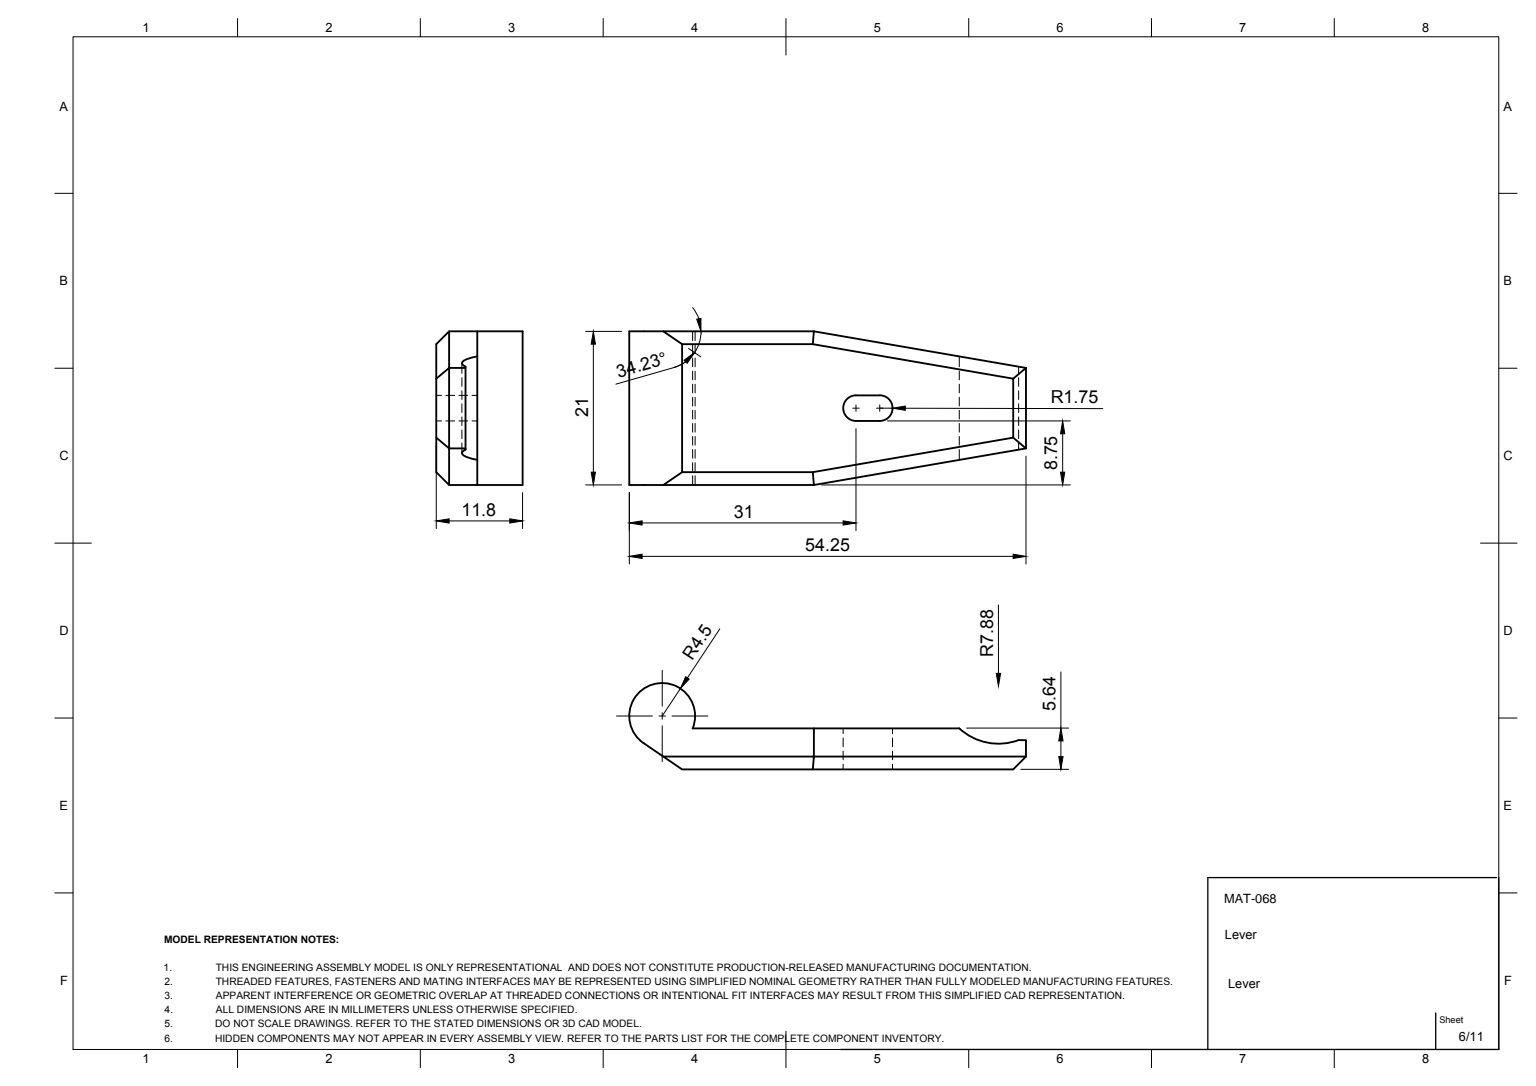
ISO-10303-21;
HEADER;
/* Generated by software containing ST-Developer
 * from STEP Tools, Inc. (www.steptools.com) 
 */

FILE_DESCRIPTION(
/* description */ ('CAx-IF Rec.Pracs.---Representation and Presentation of Product Manufa
cturing Information (PMI)---4.0---2014-10-13'),
/* implementation_level */ '2;1');

FILE_NAME(
/* name */ 'Lever.step',
/* time_stamp */ '2026-10-24T16:53:48-07:00',
/* author */ (''),
/* organization */ (''),
/* preprocessor_version */ 'ST-DEVELOPER v20.2',
/* originating_system */ 'Autodesk Translation Framework v15.17.0.0',
/* authorisation */ '');

FILE_SCHEMA (('AP242_MANAGED_MODEL_BASED_3D_ENGINEERING_MIM_LF { 1 0 10303 442 2 1 4 }'));
ENDSEC;

DATA;
#10=MECHANICAL_DESIGN_GEOMETRIC_PRESENTATION_REPRESENTATION('',(#3493),#107910);
#884=ELLIPSE('',#45698,0.00800033336362062,0.00788400944250588);
#885=ELLIPSE('',#45699,0.00800033336362222,0.0078840094425091);
#3473=SHAPE_REPRESENTATION_RELATIONSHIP('SRR','None',#107951,#3483);
#3483=ADVANCED_BREP_SHAPE_REPRESENTATION('',(#3503),#107904);
#3493=STYLED_ITEM('',(#108006),#3503);
#3503=MANIFOLD_SOLID_BREP('Body1',#45541);
#3511=FACE_BOUND('',#6702,.T.);
#3512=FACE_BOUND('',#6707,.T.);
#3550=PLANE('',#45695);
#3551=PLANE('',#45700);
#3552=PLANE('',#45701);
#3553=PLANE('',#45702);
#3554=PLANE('',#45704);
#3555=PLANE('',#45705);
#3556=PLANE('',#45706);
#3557=PLANE('',#45707);
#3558=PLANE('',#45708);
#3559=PLANE('',#45710);
#3560=PLANE('',#45711);
#3561=PLANE('',#45712);
#3562=PLANE('',#45713);
#3563=PLANE('',#45714);
#3564=PLANE('',#45715);
#3565=PLANE('',#45716);
#3773=FACE_OUTER_BOUND('',#6699,.T.);
#3774=FACE_OUTER_BOUND('',#6700,.T.);
#3775=FACE_OUTER_BOUND('',#6701,.T.);
#3776=FACE_OUTER_BOUND('',#6703,.T.);
#3777=FACE_OUTER_BOUND('',#6704,.T.);
#3778=FACE_OUTER_BOUND('',#6705,.T.);
#3779=FACE_OUTER_BOUND('',#6706,.T.);
#3780=FACE_OUTER_BOUND('',#6708,.T.);
#3781=FACE_OUTER_BOUND('',#6709,.T.);
#3782=FACE_OUTER_BOUND('',#6710,.T.);
#3783=FACE_OUTER_BOUND('',#6711,.T.);
#3784=FACE_OUTER_BOUND('',#6712,.T.);
#3785=FACE_OUTER_BOUND('',#6713,.T.);
#3786=FACE_OUTER_BOUND('',#6714,.T.);
#3787=FACE_OUTER_BOUND('',#6715,.T.);
#3788=FACE_OUTER_BOUND('',#6716,.T.);
#3789=FACE_OUTER_BOUND('',#6717,.T.);
#3790=FACE_OUTER_BOUND('',#6718,.T.);
#3791=FACE_OUTER_BOUND('',#6719,.T.);
#3792=FACE_OUTER_BOUND('',#6720,.T.);
#6699=EDGE_LOOP('',(#28164,#28165,#28166,#28167));
#6700=EDGE_LOOP('',(#28168,#28169,#28170,#28171));
#6701=EDGE_LOOP('',(#28172,#28173,#28174,#28175,#28176,#28177));
#6702=EDGE_LOOP('',(#28178,#28179,#28180,#28181));
#6703=EDGE_LOOP('',(#28182,#28183,#28184,#28185));
#6704=EDGE_LOOP('',(#28186,#28187,#28188,#28189));
#6705=EDGE_LOOP('',(#28190,#28191,#28192,#28193));
#6706=EDGE_LOOP('',(#28194,#28195,#28196,#28197,#28198,#28199));
#6707=EDGE_LOOP('',(#28200,#28201,#28202,#28203));
#6708=EDGE_LOOP('',(#28204,#28205,#28206,#28207,#28208,#28209));
#6709=EDGE_LOOP('',(#28210,#28211,#28212,#28213,#28214));
#6710=EDGE_LOOP('',(#28215,#28216,#28217,#28218,#28219));
#6711=EDGE_LOOP('',(#28220,#28221,#28222,#28223,#28224,#28225));
#6712=EDGE_LOOP('',(#28226,#28227,#28228,#28229,#28230,#28231));
#6713=EDGE_LOOP('',(#28232,#28233,#28234,#28235));
#6714=EDGE_LOOP('',(#28236,#28237,#28238,#28239));
#6715=EDGE_LOOP('',(#28240,#28241,#28242,#28243));
#6716=EDGE_LOOP('',(#28244,#28245,#28246,#28247));
#6717=EDGE_LOOP('',(#28248,#28249,#28250,#28251));
#6718=EDGE_LOOP('',(#28252,#28253,#28254,#28255));
#6719=EDGE_LOOP('',(#28256,#28257,#28258,#28259));
#6720=EDGE_LOOP('',(#28260,#28261,#28262,#28263));
#9644=LINE('',#63425,#11628);
#9645=LINE('',#63428,#11629);
#9646=LINE('',#63434,#11630);
#9647=LINE('',#63437,#11631);
#9648=LINE('',#63440,#11632);
#9649=LINE('',#63442,#11633);
#9650=LINE('',#63444,#11634);
#9651=LINE('',#63446,#11635);
#9652=LINE('',#63447,#11636);
#9653=LINE('',#63449,#11637);
#9654=LINE('',#63452,#11638);
#9655=LINE('',#63457,#11639);
#9656=LINE('',#63461,#11640);
#9657=LINE('',#63463,#11641);
#9658=LINE('',#63464,#11642);
#9659=LINE('',#63467,#11643);
#9660=LINE('',#63469,#11644);
#9661=LINE('',#63470,#11645);
#9662=LINE('',#63474,#11646);
#9663=LINE('',#63476,#11647);
#9664=LINE('',#63478,#11648);
#9665=LINE('',#63480,#11649);
#9666=LINE('',#63482,#11650);
#9667=LINE('',#63483,#11651);
#9668=LINE('',#63485,#11652);
#9669=LINE('',#63488,#11653);
#9670=LINE('',#63491,#11654);
#9671=LINE('',#63492,#11655);
#9672=LINE('',#63494,#11656);
#9673=LINE('',#63495,#11657);
#9674=LINE('',#63498,#11658);
#9675=LINE('',#63499,#11659);
#9676=LINE('',#63502,#11660);
#9677=LINE('',#63503,#11661);
#9678=LINE('',#63505,#11662);
#9679=LINE('',#63507,#11663);
#9680=LINE('',#63509,#11664);
#9681=LINE('',#63510,#11665);
#9682=LINE('',#63514,#11666);
#9683=LINE('',#63516,#11667);
#9684=LINE('',#63518,#11668);
#9685=LINE('',#63520,#11669);
#11628=VECTOR('',#50447,1.);
#11629=VECTOR('',#50450,1.);
#11630=VECTOR('',#50455,1.);
#11631=VECTOR('',#50458,1.);
#11632=VECTOR('',#50461,1.);
#11633=VECTOR('',#50462,1.);
#11634=VECTOR('',#50463,1.);
#11635=VECTOR('',#50464,1.);
#11636=VECTOR('',#50465,1.);
#11637=VECTOR('',#50466,1.);
#11638=VECTOR('',#50469,1.);
#11639=VECTOR('',#50474,1.);
#11640=VECTOR('',#50479,1.);
#11641=VECTOR('',#50480,1.);
#11642=VECTOR('',#50481,1.);
#11643=VECTOR('',#50484,1.);
#11644=VECTOR('',#50485,1.);
#11645=VECTOR('',#50486,1.);
#11646=VECTOR('',#50489,1.);
#11647=VECTOR('',#50490,1.);
#11648=VECTOR('',#50491,1.);
#11649=VECTOR('',#50492,1.);
#11650=VECTOR('',#50493,1.);
#11651=VECTOR('',#50494,1.);
#11652=VECTOR('',#50495,1.);
#11653=VECTOR('',#50498,1.);
#11654=VECTOR('',#50501,1.);
#11655=VECTOR('',#50502,1.);
#11656=VECTOR('',#50503,1.);
#11657=VECTOR('',#50504,1.);
#11658=VECTOR('',#50507,1.);
#11659=VECTOR('',#50508,1.);
#11660=VECTOR('',#50511,1.);
#11661=VECTOR('',#50512,1.);
#11662=VECTOR('',#50515,1.);
#11663=VECTOR('',#50518,1.);
#11664=VECTOR('',#50521,1.);
#11665=VECTOR('',#50522,1.);
#11666=VECTOR('',#50529,1.);
#11667=VECTOR('',#50532,1.);
#11668=VECTOR('',#50535,1.);
#11669=VECTOR('',#50538,1.);
#13618=CIRCLE('',#45690,0.00175000000001001);
#13619=CIRCLE('',#45691,0.00175000000001001);
#13620=CIRCLE('',#45693,0.00450000000001);
#13621=CIRCLE('',#45694,0.00450000000001);
#13622=CIRCLE('',#45696,0.00175000000001001);
#13623=CIRCLE('',#45703,0.00175000000001001);
#17193=VERTEX_POINT('',#63421);
#17194=VERTEX_POINT('',#63422);
#17195=VERTEX_POINT('',#63424);
#17196=VERTEX_POINT('',#63426);
#17197=VERTEX_POINT('',#63430);
#17198=VERTEX_POINT('',#63431);
#17199=VERTEX_POINT('',#63433);
#17200=VERTEX_POINT('',#63435);
#17201=VERTEX_POINT('',#63439);
#17202=VERTEX_POINT('',#63441);
#17203=VERTEX_POINT('',#63443);
#17204=VERTEX_POINT('',#63445);
#17205=VERTEX_POINT('',#63448);
#17206=VERTEX_POINT('',#63450);
#17207=VERTEX_POINT('',#63454);
#17208=VERTEX_POINT('',#63456);
#17209=VERTEX_POINT('',#63460);
#17210=VERTEX_POINT('',#63462);
#17211=VERTEX_POINT('',#63466);
#17212=VERTEX_POINT('',#63468);
#17213=VERTEX_POINT('',#63472);
#17214=VERTEX_POINT('',#63473);
#17215=VERTEX_POINT('',#63475);
#17216=VERTEX_POINT('',#63477);
#17217=VERTEX_POINT('',#63479);
#17218=VERTEX_POINT('',#63481);
#17219=VERTEX_POINT('',#63484);
#17220=VERTEX_POINT('',#63486);
#17221=VERTEX_POINT('',#63490);
#17222=VERTEX_POINT('',#63493);
#17223=VERTEX_POINT('',#63497);
#17224=VERTEX_POINT('',#63501);
#21224=EDGE_CURVE('',#17193,#17194,#13618,.T.);
#21225=EDGE_CURVE('',#17194,#17195,#9644,.T.);
#21226=EDGE_CURVE('',#17195,#17196,#13619,.T.);
#21227=EDGE_CURVE('',#17193,#17196,#9645,.T.);
#21228=EDGE_CURVE('',#17197,#17198,#13620,.T.);
#21229=EDGE_CURVE('',#17197,#17199,#9646,.T.);
#21230=EDGE_CURVE('',#17199,#17200,#13621,.T.);
#21231=EDGE_CURVE('',#17198,#17200,#9647,.T.);
#21232=EDGE_CURVE('',#17200,#17201,#9648,.T.);
#21233=EDGE_CURVE('',#17202,#17201,#9649,.T.);
#21234=EDGE_CURVE('',#17203,#17202,#9650,.T.);
#21235=EDGE_CURVE('',#17204,#17203,#9651,.T.);
#21236=EDGE_CURVE('',#17198,#17204,#9652,.T.);
#21237=EDGE_CURVE('',#17205,#17193,#9653,.T.);
#21238=EDGE_CURVE('',#17206,#17205,#13622,.T.);
#21239=EDGE_CURVE('',#17194,#17206,#9654,.T.);
#21240=EDGE_CURVE('',#17202,#17207,#884,.T.);
#21241=EDGE_CURVE('',#17208,#17207,#9655,.T.);
#21242=EDGE_CURVE('',#17208,#17203,#885,.T.);
#21243=EDGE_CURVE('',#17207,#17209,#9656,.T.);
#21244=EDGE_CURVE('',#17210,#17209,#9657,.T.);
#21245=EDGE_CURVE('',#17210,#17208,#9658,.T.);
#21246=EDGE_CURVE('',#17209,#17211,#9659,.T.);
#21247=EDGE_CURVE('',#17211,#17212,#9660,.T.);
#21248=EDGE_CURVE('',#17210,#17212,#9661,.T.);
#21249=EDGE_CURVE('',#17213,#17214,#9662,.T.);
#21250=EDGE_CURVE('',#17214,#17215,#9663,.T.);
#21251=EDGE_CURVE('',#17216,#17215,#9664,.T.);
#21252=EDGE_CURVE('',#17216,#17217,#9665,.T.);
#21253=EDGE_CURVE('',#17217,#17218,#9666,.T.);
#21254=EDGE_CURVE('',#17218,#17213,#9667,.T.);
#21255=EDGE_CURVE('',#17219,#17195,#9668,.T.);
#21256=EDGE_CURVE('',#17220,#17219,#13623,.T.);
#21257=EDGE_CURVE('',#17196,#17220,#9669,.T.);
#21258=EDGE_CURVE('',#17215,#17221,#9670,.T.);
#21259=EDGE_CURVE('',#17221,#17199,#9671,.T.);
#21260=EDGE_CURVE('',#17222,#17197,#9672,.T.);
#21261=EDGE_CURVE('',#17222,#17216,#9673,.T.);
#21262=EDGE_CURVE('',#17204,#17223,#9674,.T.);
#21263=EDGE_CURVE('',#17223,#17222,#9675,.T.);
#21264=EDGE_CURVE('',#17221,#17224,#9676,.T.);
#21265=EDGE_CURVE('',#17201,#17224,#9677,.T.);
#21266=EDGE_CURVE('',#17224,#17211,#9678,.T.);
#21267=EDGE_CURVE('',#17212,#17223,#9679,.T.);
#21268=EDGE_CURVE('',#17205,#17220,#9680,.T.);
#21269=EDGE_CURVE('',#17206,#17219,#9681,.T.);
#21270=EDGE_CURVE('',#17217,#17223,#9682,.T.);
#21271=EDGE_CURVE('',#17218,#17212,#9683,.T.);
#21272=EDGE_CURVE('',#17213,#17211,#9684,.T.);
#21273=EDGE_CURVE('',#17214,#17224,#9685,.T.);
#28164=ORIENTED_EDGE('',*,*,#21224,.T.);
#28165=ORIENTED_EDGE('',*,*,#21225,.T.);
#28166=ORIENTED_EDGE('',*,*,#21226,.T.);
#28167=ORIENTED_EDGE('',*,*,#21227,.F.);
#28168=ORIENTED_EDGE('',*,*,#21228,.F.);
#28169=ORIENTED_EDGE('',*,*,#21229,.T.);
#28170=ORIENTED_EDGE('',*,*,#21230,.T.);
#28171=ORIENTED_EDGE('',*,*,#21231,.F.);
#28172=ORIENTED_EDGE('',*,*,#21232,.T.);
#28173=ORIENTED_EDGE('',*,*,#21233,.F.);
#28174=ORIENTED_EDGE('',*,*,#21234,.F.);
#28175=ORIENTED_EDGE('',*,*,#21235,.F.);
#28176=ORIENTED_EDGE('',*,*,#21236,.F.);
#28177=ORIENTED_EDGE('',*,*,#21231,.T.);
#28178=ORIENTED_EDGE('',*,*,#21237,.F.);
#28179=ORIENTED_EDGE('',*,*,#21238,.F.);
#28180=ORIENTED_EDGE('',*,*,#21239,.F.);
#28181=ORIENTED_EDGE('',*,*,#21224,.F.);
#28182=ORIENTED_EDGE('',*,*,#21234,.T.);
#28183=ORIENTED_EDGE('',*,*,#21240,.T.);
#28184=ORIENTED_EDGE('',*,*,#21241,.F.);
#28185=ORIENTED_EDGE('',*,*,#21242,.T.);
#28186=ORIENTED_EDGE('',*,*,#21241,.T.);
#28187=ORIENTED_EDGE('',*,*,#21243,.T.);
#28188=ORIENTED_EDGE('',*,*,#21244,.F.);
#28189=ORIENTED_EDGE('',*,*,#21245,.T.);
#28190=ORIENTED_EDGE('',*,*,#21246,.T.);
#28191=ORIENTED_EDGE('',*,*,#21247,.T.);
#28192=ORIENTED_EDGE('',*,*,#21248,.F.);
#28193=ORIENTED_EDGE('',*,*,#21244,.T.);
#28194=ORIENTED_EDGE('',*,*,#21249,.T.);
#28195=ORIENTED_EDGE('',*,*,#21250,.T.);
#28196=ORIENTED_EDGE('',*,*,#21251,.F.);
#28197=ORIENTED_EDGE('',*,*,#21252,.T.);
#28198=ORIENTED_EDGE('',*,*,#21253,.T.);
#28199=ORIENTED_EDGE('',*,*,#21254,.T.);
#28200=ORIENTED_EDGE('',*,*,#21255,.F.);
#28201=ORIENTED_EDGE('',*,*,#21256,.F.);
#28202=ORIENTED_EDGE('',*,*,#21257,.F.);
#28203=ORIENTED_EDGE('',*,*,#21226,.F.);
#28204=ORIENTED_EDGE('',*,*,#21251,.T.);
#28205=ORIENTED_EDGE('',*,*,#21258,.T.);
#28206=ORIENTED_EDGE('',*,*,#21259,.T.);
#28207=ORIENTED_EDGE('',*,*,#21229,.F.);
#28208=ORIENTED_EDGE('',*,*,#21260,.F.);
#28209=ORIENTED_EDGE('',*,*,#21261,.T.);
#28210=ORIENTED_EDGE('',*,*,#21262,.T.);
#28211=ORIENTED_EDGE('',*,*,#21263,.T.);
#28212=ORIENTED_EDGE('',*,*,#21260,.T.);
#28213=ORIENTED_EDGE('',*,*,#21228,.T.);
#28214=ORIENTED_EDGE('',*,*,#21236,.T.);
#28215=ORIENTED_EDGE('',*,*,#21259,.F.);
#28216=ORIENTED_EDGE('',*,*,#21264,.T.);
#28217=ORIENTED_EDGE('',*,*,#21265,.F.);
#28218=ORIENTED_EDGE('',*,*,#21232,.F.);
#28219=ORIENTED_EDGE('',*,*,#21230,.F.);
#28220=ORIENTED_EDGE('',*,*,#21265,.T.);
#28221=ORIENTED_EDGE('',*,*,#21266,.T.);
#28222=ORIENTED_EDGE('',*,*,#21246,.F.);
#28223=ORIENTED_EDGE('',*,*,#21243,.F.);
#28224=ORIENTED_EDGE('',*,*,#21240,.F.);
#28225=ORIENTED_EDGE('',*,*,#21233,.T.);
#28226=ORIENTED_EDGE('',*,*,#21248,.T.);
#28227=ORIENTED_EDGE('',*,*,#21267,.T.);
#28228=ORIENTED_EDGE('',*,*,#21262,.F.);
#28229=ORIENTED_EDGE('',*,*,#21235,.T.);
#28230=ORIENTED_EDGE('',*,*,#21242,.F.);
#28231=ORIENTED_EDGE('',*,*,#21245,.F.);
#28232=ORIENTED_EDGE('',*,*,#21238,.T.);
#28233=ORIENTED_EDGE('',*,*,#21268,.T.);
#28234=ORIENTED_EDGE('',*,*,#21256,.T.);
#28235=ORIENTED_EDGE('',*,*,#21269,.F.);
#28236=ORIENTED_EDGE('',*,*,#21237,.T.);
#28237=ORIENTED_EDGE('',*,*,#21227,.T.);
#28238=ORIENTED_EDGE('',*,*,#21257,.T.);
#28239=ORIENTED_EDGE('',*,*,#21268,.F.);
#28240=ORIENTED_EDGE('',*,*,#21239,.T.);
#28241=ORIENTED_EDGE('',*,*,#21269,.T.);
#28242=ORIENTED_EDGE('',*,*,#21255,.T.);
#28243=ORIENTED_EDGE('',*,*,#21225,.F.);
#28244=ORIENTED_EDGE('',*,*,#21261,.F.);
#28245=ORIENTED_EDGE('',*,*,#21263,.F.);
#28246=ORIENTED_EDGE('',*,*,#21270,.F.);
#28247=ORIENTED_EDGE('',*,*,#21252,.F.);
#28248=ORIENTED_EDGE('',*,*,#21270,.T.);
#28249=ORIENTED_EDGE('',*,*,#21267,.F.);
#28250=ORIENTED_EDGE('',*,*,#21271,.F.);
#28251=ORIENTED_EDGE('',*,*,#21253,.F.);
#28252=ORIENTED_EDGE('',*,*,#21271,.T.);
#28253=ORIENTED_EDGE('',*,*,#21247,.F.);
#28254=ORIENTED_EDGE('',*,*,#21272,.F.);
#28255=ORIENTED_EDGE('',*,*,#21254,.F.);
#28256=ORIENTED_EDGE('',*,*,#21272,.T.);
#28257=ORIENTED_EDGE('',*,*,#21266,.F.);
#28258=ORIENTED_EDGE('',*,*,#21273,.F.);
#28259=ORIENTED_EDGE('',*,*,#21249,.F.);
#28260=ORIENTED_EDGE('',*,*,#21273,.T.);
#28261=ORIENTED_EDGE('',*,*,#21264,.F.);
#28262=ORIENTED_EDGE('',*,*,#21258,.F.);
#28263=ORIENTED_EDGE('',*,*,#21250,.F.);
#41965=CYLINDRICAL_SURFACE('',#45689,0.00175);
#41966=CYLINDRICAL_SURFACE('',#45692,0.0045);
#41967=CYLINDRICAL_SURFACE('',#45697,0.00788400944250797);
#41968=CYLINDRICAL_SURFACE('',#45709,0.00175);
#42628=ADVANCED_FACE('',(#3773),#41965,.F.);
#42629=ADVANCED_FACE('',(#3774),#41966,.T.);
#42630=ADVANCED_FACE('',(#3775,#3511),#3550,.F.);
#42631=ADVANCED_FACE('',(#3776),#41967,.F.);
#42632=ADVANCED_FACE('',(#3777),#3551,.F.);
#42633=ADVANCED_FACE('',(#3778),#3552,.F.);
#42634=ADVANCED_FACE('',(#3779,#3512),#3553,.F.);
#42635=ADVANCED_FACE('',(#3780),#3554,.F.);
#42636=ADVANCED_FACE('',(#3781),#3555,.T.);
#42637=ADVANCED_FACE('',(#3782),#3556,.T.);
#42638=ADVANCED_FACE('',(#3783),#3557,.F.);
#42639=ADVANCED_FACE('',(#3784),#3558,.F.);
#42640=ADVANCED_FACE('',(#3785),#41968,.F.);
#42641=ADVANCED_FACE('',(#3786),#3559,.F.);
#42642=ADVANCED_FACE('',(#3787),#3560,.F.);
#42643=ADVANCED_FACE('',(#3788),#3561,.T.);
#42644=ADVANCED_FACE('',(#3789),#3562,.F.);
#42645=ADVANCED_FACE('',(#3790),#3563,.F.);
#42646=ADVANCED_FACE('',(#3791),#3564,.F.);
#42647=ADVANCED_FACE('',(#3792),#3565,.T.);
#45541=CLOSED_SHELL('',(#42628,#42629,#42630,#42631,#42632,#42633,#42634,
#42635,#42636,#42637,#42638,#42639,#42640,#42641,#42642,#42643,#42644,#42645,
#42646,#42647));
#45688=AXIS2_PLACEMENT_3D('',#63419,#50441,#50442);
#45689=AXIS2_PLACEMENT_3D('',#63420,#50443,#50444);
#45690=AXIS2_PLACEMENT_3D('',#63423,#50445,#50446);
#45691=AXIS2_PLACEMENT_3D('',#63427,#50448,#50449);
#45692=AXIS2_PLACEMENT_3D('',#63429,#50451,#50452);
#45693=AXIS2_PLACEMENT_3D('',#63432,#50453,#50454);
#45694=AXIS2_PLACEMENT_3D('',#63436,#50456,#50457);
#45695=AXIS2_PLACEMENT_3D('',#63438,#50459,#50460);
#45696=AXIS2_PLACEMENT_3D('',#63451,#50467,#50468);
#45697=AXIS2_PLACEMENT_3D('',#63453,#50470,#50471);
#45698=AXIS2_PLACEMENT_3D('',#63455,#50472,#50473);
#45699=AXIS2_PLACEMENT_3D('',#63458,#50475,#50476);
#45700=AXIS2_PLACEMENT_3D('',#63459,#50477,#50478);
#45701=AXIS2_PLACEMENT_3D('',#63465,#50482,#50483);
#45702=AXIS2_PLACEMENT_3D('',#63471,#50487,#50488);
#45703=AXIS2_PLACEMENT_3D('',#63487,#50496,#50497);
#45704=AXIS2_PLACEMENT_3D('',#63489,#50499,#50500);
#45705=AXIS2_PLACEMENT_3D('',#63496,#50505,#50506);
#45706=AXIS2_PLACEMENT_3D('',#63500,#50509,#50510);
#45707=AXIS2_PLACEMENT_3D('',#63504,#50513,#50514);
#45708=AXIS2_PLACEMENT_3D('',#63506,#50516,#50517);
#45709=AXIS2_PLACEMENT_3D('',#63508,#50519,#50520);
#45710=AXIS2_PLACEMENT_3D('',#63511,#50523,#50524);
#45711=AXIS2_PLACEMENT_3D('',#63512,#50525,#50526);
#45712=AXIS2_PLACEMENT_3D('',#63513,#50527,#50528);
#45713=AXIS2_PLACEMENT_3D('',#63515,#50530,#50531);
#45714=AXIS2_PLACEMENT_3D('',#63517,#50533,#50534);
#45715=AXIS2_PLACEMENT_3D('',#63519,#50536,#50537);
#45716=AXIS2_PLACEMENT_3D('',#63521,#50539,#50540);
#50441=DIRECTION('axis',(0.,0.,1.));
#50442=DIRECTION('refdir',(1.,0.,0.));
#50443=DIRECTION('center_axis',(0.,-1.,1.45983193964168E-32));
#50444=DIRECTION('ref_axis',(1.,0.,0.));
#50445=DIRECTION('center_axis',(0.,1.,-5.71428571425305E-12));
#50446=DIRECTION('ref_axis',(1.,0.,0.));
#50447=DIRECTION('',(-1.01199007411378E-14,-1.,1.E-14));
#50448=DIRECTION('center_axis',(0.,-1.,5.71428571425305E-12));
#50449=DIRECTION('ref_axis',(1.,0.,0.));
#50450=DIRECTION('',(-1.01199007411378E-14,-1.,1.E-14));
#50451=DIRECTION('center_axis',(0.,8.34284178923119E-33,1.));
#50452=DIRECTION('ref_axis',(-0.288781765961724,0.95739495071158,-7.9873946035955E-33));
#50453=DIRECTION('center_axis',(0.,0.,-1.));
#50454=DIRECTION('ref_axis',(-1.,0.,0.));
#50455=DIRECTION('',(1.00521721346157E-14,1.E-14,1.));
#50456=DIRECTION('center_axis',(0.,-2.22222222221729E-12,-1.));
#50457=DIRECTION('ref_axis',(1.,0.,0.));
#50458=DIRECTION('',(1.00521721346157E-14,1.E-14,1.));
#50459=DIRECTION('center_axis',(1.18937267665668E-17,-1.,7.7223206752818E-33));
#50460=DIRECTION('ref_axis',(-7.5891469116954E-66,-7.7223206752818E-33,
-1.));
#50461=DIRECTION('',(1.,1.00118937267665E-14,-1.02086885384633E-14));
#50462=DIRECTION('',(-0.985460115744347,-1.00117207933559E-14,0.169906916507654));
#50463=DIRECTION('',(1.00521721346157E-14,1.E-14,1.));
#50464=DIRECTION('',(0.985460115744347,1.00117207933559E-14,0.169906916507654));
#50465=DIRECTION('',(1.,1.00118937267665E-14,0.));
#50466=DIRECTION('',(1.,1.00118937267665E-14,-1.E-14));
#50467=DIRECTION('center_axis',(0.,1.,-5.71428571425305E-12));
#50468=DIRECTION('ref_axis',(1.,0.,0.));
#50469=DIRECTION('',(-1.,-1.00118937267665E-14,1.E-14));
#50470=DIRECTION('center_axis',(0.,8.34284178923119E-33,1.));
#50471=DIRECTION('ref_axis',(1.,0.,0.));
#50472=DIRECTION('center_axis',(0.169906916507649,2.14440522290675E-14,
0.985460115744348));
#50473=DIRECTION('ref_axis',(0.985460115744348,-2.65533858744027E-12,-0.169906916507649));
#50474=DIRECTION('',(1.00521721346157E-14,1.E-14,1.));
#50475=DIRECTION('center_axis',(0.169906916507651,-2.62034553422522E-14,
-0.985460115744347));
#50476=DIRECTION('ref_axis',(-0.985460115744347,-7.81400541235329E-14,-0.169906916507651));
#50477=DIRECTION('center_axis',(0.,-1.,8.34284178923119E-33));
#50478=DIRECTION('ref_axis',(-1.,0.,0.));
#50479=DIRECTION('',(0.985460115744347,-9.99999999999989E-15,-0.169906916507654));
#50480=DIRECTION('',(1.00521721346157E-14,1.E-14,1.));
#50481=DIRECTION('',(-0.985460115744347,-9.99999999999989E-15,-0.169906916507654));
#50482=DIRECTION('center_axis',(-1.,0.,5.21721346158438E-17));
#50483=DIRECTION('ref_axis',(0.,1.,0.));
#50484=DIRECTION('',(-1.01199007411378E-14,-1.,1.E-14));
#50485=DIRECTION('',(-1.00521721346157E-14,-1.E-14,-1.));
#50486=DIRECTION('',(-1.01199007411378E-14,-1.,1.E-14));
#50487=DIRECTION('center_axis',(-2.66337519831924E-50,1.,-2.22131671000782E-34));
#50488=DIRECTION('ref_axis',(1.,2.37389193643995E-65,-1.19900741137893E-16));
#50489=DIRECTION('',(-0.985460115744347,1.01181573982395E-14,0.169906916507654));
#50490=DIRECTION('',(-1.,1.01199007411378E-14,1.02086885384633E-14));
#50491=DIRECTION('',(1.00521721346157E-14,1.E-14,1.));
#50492=DIRECTION('',(1.,-1.01199007411378E-14,0.));
#50493=DIRECTION('',(0.985460115744347,-1.01181573982395E-14,0.169906916507654));
#50494=DIRECTION('',(1.00521721346157E-14,1.E-14,1.));
#50495=DIRECTION('',(1.,-1.01334402673827E-14,0.));
#50496=DIRECTION('center_axis',(0.,-1.,5.71428571425305E-12));
#50497=DIRECTION('ref_axis',(1.,0.,0.));
#50498=DIRECTION('',(-1.,1.01334402673827E-14,0.));
#50499=DIRECTION('center_axis',(0.562571578885413,0.8267485824786,-2.93505601446575E-17));
#50500=DIRECTION('ref_axis',(-5.21721346158438E-17,6.35926162475305E-32,
-1.));
#50501=DIRECTION('',(-0.72055180024015,0.490308628911769,0.490308628911771));
#50502=DIRECTION('',(-0.826748582478598,0.562571578885415,1.0172532953354E-14));
#50503=DIRECTION('',(-0.826748582478598,0.562571578885415,0.));
#50504=DIRECTION('',(0.720551800240151,-0.490308628911769,0.49030862891177));
#50505=DIRECTION('center_axis',(0.,0.,-1.));
#50506=DIRECTION('ref_axis',(0.,-1.,0.));
#50507=DIRECTION('',(-1.01199007411378E-14,-1.,1.E-14));
#50508=DIRECTION('',(-1.,1.01199007411378E-14,0.));
#50509=DIRECTION('center_axis',(1.60527967783421E-47,7.69222732429044E-32,
1.));
#50510=DIRECTION('ref_axis',(1.,-2.08688538463375E-16,-3.50729211666941E-63));
#50511=DIRECTION('',(1.,-1.01199007411378E-14,-1.02086885384633E-14));
#50512=DIRECTION('',(-1.01199007411378E-14,-1.,1.E-14));
#50513=DIRECTION('center_axis',(-0.169906916507646,2.03719652137209E-17,
-0.985460115744348));
#50514=DIRECTION('ref_axis',(-0.985460115744348,-9.68087878944276E-35,0.169906916507646));
#50515=DIRECTION('',(0.985460115744347,-1.01181573982395E-14,-0.169906916507654));
#50516=DIRECTION('center_axis',(-0.169906916507646,2.03719652137209E-17,
0.985460115744348));
#50517=DIRECTION('ref_axis',(1.19900741137893E-16,1.,-3.62640108812244E-32));
#50518=DIRECTION('',(-0.985460115744347,1.01181573982395E-14,-0.169906916507654));
#50519=DIRECTION('center_axis',(0.,-1.,1.45983193964168E-32));
#50520=DIRECTION('ref_axis',(-1.,1.78777851217525E-48,1.22464679914735E-16));
#50521=DIRECTION('',(-1.01199007411378E-14,-1.,1.E-14));
#50522=DIRECTION('',(-1.01199007411378E-14,-1.,1.E-14));
#50523=DIRECTION('center_axis',(2.84375793746248E-80,1.45983193964168E-32,
1.));
#50524=DIRECTION('ref_axis',(1.,-1.94800364359783E-48,8.31581056687692E-97));
#50525=DIRECTION('center_axis',(-1.94800364359783E-48,-1.45983193964168E-32,
-1.));
#50526=DIRECTION('ref_axis',(0.,-1.,1.45983193964168E-32));
#50527=DIRECTION('center_axis',(-8.47826271278967E-17,-0.707106781186549,
-0.707106781186547));
#50528=DIRECTION('ref_axis',(-1.48909625690539E-32,0.707106781186547,-0.707106781186549));
#50529=DIRECTION('',(0.060400598363751,0.705815757729061,-0.705815757729064));
#50530=DIRECTION('center_axis',(-0.120142332833053,0.707106781186551,0.696825530431705));
#50531=DIRECTION('ref_axis',(0.985460115744348,6.9160230078685E-16,0.169906916507646));
#50532=DIRECTION('',(0.607508557019365,0.60750855701936,-0.511729133718712));
#50533=DIRECTION('center_axis',(-0.707106781186545,0.707106781186551,3.68912701758404E-17));
#50534=DIRECTION('ref_axis',(5.21721346158438E-17,4.12364695333908E-32,
1.));
#50535=DIRECTION('',(0.607508557019368,0.607508557019363,0.511729133718706));
#50536=DIRECTION('center_axis',(-0.120142332833053,0.707106781186546,-0.69682553043171));
#50537=DIRECTION('ref_axis',(-0.985460115744348,3.52718437708667E-16,0.169906916507646));
#50538=DIRECTION('',(0.0604005983636862,0.705815757729064,0.705815757729067));
#50539=DIRECTION('center_axis',(6.27824535754649E-17,-0.707106781186549,
0.707106781186546));
#50540=DIRECTION('ref_axis',(-1.,-8.87877973254815E-17,-2.5390518211582E-32));
#63419=CARTESIAN_POINT('',(0.,0.,0.));
#63420=CARTESIAN_POINT('Origin',(0.0111237821931084,0.0230268185280382,
0.07415));
#63421=CARTESIAN_POINT('',(0.0111237821931084,-0.0145741814719618,0.0759));
#63422=CARTESIAN_POINT('',(0.0111237821931084,-0.0145741814719618,0.0724));
#63423=CARTESIAN_POINT('Origin',(0.0111237821931184,-0.0145741814719718,
0.07415000000001));
#63424=CARTESIAN_POINT('',(0.0111237821931084,-0.0201741814719619,0.0724));
#63425=CARTESIAN_POINT('',(0.0111237821931184,0.0230268185280482,0.07240000000001));
#63426=CARTESIAN_POINT('',(0.0111237821931084,-0.0201741814719619,0.0759));
#63427=CARTESIAN_POINT('Origin',(0.0111237821931184,-0.0201741814719718,
0.07415000000001));
#63428=CARTESIAN_POINT('',(0.0111237821931184,0.0230268185280482,0.07590000000001));
#63429=CARTESIAN_POINT('Origin',(-0.0186262178068916,-0.0128741814719618,
0.00803151208831422));
#63430=CARTESIAN_POINT('',(-0.0211577899118759,-0.0165945500931155,0.06365));
#63431=CARTESIAN_POINT('',(-0.0144596844756917,-0.0145741814719618,0.06365));
#63432=CARTESIAN_POINT('Origin',(-0.0186262178069016,-0.0128741814719718,
0.06365000000001));
#63433=CARTESIAN_POINT('',(-0.0211577899118759,-0.0165945500931155,0.08465));
#63434=CARTESIAN_POINT('',(-0.0211577899118859,-0.0165945500931255,0.00803151208832422));
#63435=CARTESIAN_POINT('',(-0.0144596844756917,-0.0145741814719618,0.08465));
#63436=CARTESIAN_POINT('Origin',(-0.0186262178069016,-0.0128741814719718,
0.08465000000001));
#63437=CARTESIAN_POINT('',(-0.0144596844757017,-0.0145741814719718,0.00803151208832422));
#63438=CARTESIAN_POINT('Origin',(0.0220033079492963,-0.0145741814719618,
0.00803151208831422));
#63439=CARTESIAN_POINT('',(0.0021237821931084,-0.0145741814719618,0.08465));
#63440=CARTESIAN_POINT('',(0.0220033079493063,-0.0145741814719718,0.08465000000001));
#63441=CARTESIAN_POINT('',(0.0220033079492963,-0.0145741814719618,0.0812224955592779));
#63442=CARTESIAN_POINT('',(0.00212378219311841,-0.0145741814719718,0.08465000000001));
#63443=CARTESIAN_POINT('',(0.0220033079492963,-0.0145741814719618,0.067077504440722));
#63444=CARTESIAN_POINT('',(0.0220033079493063,-0.0145741814719718,0.00803151208832422));
#63445=CARTESIAN_POINT('',(0.0021237821931084,-0.0145741814719618,0.06365));
#63446=CARTESIAN_POINT('',(0.0311237821931184,-0.0145741814719718,0.06865000000001));
#63447=CARTESIAN_POINT('',(0.0220033079493063,-0.0145741814719718,0.06365000000001));
#63448=CARTESIAN_POINT('',(0.0078737821931084,-0.0145741814719618,0.0759));
#63449=CARTESIAN_POINT('',(0.00787378219311841,-0.0145741814719718,0.07590000000001));
#63450=CARTESIAN_POINT('',(0.0078737821931084,-0.0145741814719618,0.0724));
#63451=CARTESIAN_POINT('Origin',(0.0078737821931184,-0.0145741814719718,
0.07415000000001));
#63452=CARTESIAN_POINT('',(0.00787378219311841,-0.0145741814719718,0.07240000000001));
#63453=CARTESIAN_POINT('Origin',(0.0273608110672173,-0.00879017202945387,
0.00803151208831422));
#63454=CARTESIAN_POINT('',(0.0301237821931084,-0.0161741814719619,0.0798224137931034));
#63455=CARTESIAN_POINT('Origin',(0.0273608110672267,-0.00879017202946598,
0.0802987881251636));
#63456=CARTESIAN_POINT('',(0.0301237821931084,-0.0161741814719619,0.0684775862068966));
#63457=CARTESIAN_POINT('',(0.0301237821931184,-0.0161741814719718,0.00803151208832422));
#63458=CARTESIAN_POINT('Origin',(0.0273608110672274,-0.00879017202946274,
0.0680012118748562));
#63459=CARTESIAN_POINT('Origin',(0.0311237821931084,-0.0161741814719619,
0.00803151208831422));
#63460=CARTESIAN_POINT('',(0.0311237821931084,-0.0161741814719619,0.07965));
#63461=CARTESIAN_POINT('',(0.0431153304000404,-0.0161741814719718,0.0775824916884717));
#63462=CARTESIAN_POINT('',(0.0311237821931084,-0.0161741814719619,0.06865));
#63463=CARTESIAN_POINT('',(0.0311237821931184,-0.0161741814719718,0.00803151208832422));
#63464=CARTESIAN_POINT('',(0.0209740353718777,-0.0161741814719718,0.0669000436515202));
#63465=CARTESIAN_POINT('Origin',(0.0311237821931084,-0.0201741814719619,
0.00803151208831422));
#63466=CARTESIAN_POINT('',(0.0311237821931084,-0.0184241814719618,0.07965));
#63467=CARTESIAN_POINT('',(0.0311237821931184,0.0148536964671725,0.07965000000001));
#63468=CARTESIAN_POINT('',(0.0311237821931084,-0.0184241814719618,0.06865));
#63469=CARTESIAN_POINT('',(0.0311237821931184,-0.0184241814719718,0.00803151208832422));
#63470=CARTESIAN_POINT('',(0.0311237821931184,0.0148536964671725,0.06865000000001));
#63471=CARTESIAN_POINT('Origin',(-0.0158972056958719,-0.0201741814719619,
0.00803151208831422));
#63472=CARTESIAN_POINT('',(0.0293737821931084,-0.0201741814719619,0.0781759039174667));
#63473=CARTESIAN_POINT('',(0.001974024914415,-0.0201741814719619,0.0829));
#63474=CARTESIAN_POINT('',(-0.00284557577388231,-0.0201741814719718,0.0837309656359216));
#63475=CARTESIAN_POINT('',(-0.0158972056958719,-0.0201741814719619,0.0829));
#63476=CARTESIAN_POINT('',(-0.0158972056958819,-0.0201741814719718,0.08290000000001));
#63477=CARTESIAN_POINT('',(-0.0158972056958719,-0.0201741814719619,0.0654));
#63478=CARTESIAN_POINT('',(-0.0158972056958819,-0.0201741814719718,0.00803151208832422));
#63479=CARTESIAN_POINT('',(0.00197402491441486,-0.0201741814719619,0.0654));
#63480=CARTESIAN_POINT('',(0.0021237821931184,-0.0201741814719718,0.06540000000001));
#63481=CARTESIAN_POINT('',(0.0293737821931084,-0.0201741814719619,0.0701240960825334));
#63482=CARTESIAN_POINT('',(-0.024986870802045,-0.0201741814719718,0.0607515697040704));
#63483=CARTESIAN_POINT('',(0.0293737821931184,-0.0201741814719718,0.00803151208832422));
#63484=CARTESIAN_POINT('',(0.0078737821931084,-0.0201741814719619,0.0724));
#63485=CARTESIAN_POINT('',(0.0078737821931184,-0.0201741814719718,0.07240000000001));
#63486=CARTESIAN_POINT('',(0.0078737821931084,-0.0201741814719619,0.0759));
#63487=CARTESIAN_POINT('Origin',(0.0078737821931184,-0.0201741814719718,
0.07415000000001));
#63488=CARTESIAN_POINT('',(0.0078737821931184,-0.0201741814719718,0.07590000000001));
#63489=CARTESIAN_POINT('Origin',(-0.0211577899118759,-0.0165945500931155,
0.00803151208831422));
#63490=CARTESIAN_POINT('',(-0.0184689851345062,-0.0184241814719618,0.08465));
#63491=CARTESIAN_POINT('',(-0.0158972056958818,-0.0201741814719718,0.08290000000001));
#63492=CARTESIAN_POINT('',(-0.0211577899118859,-0.0165945500931255,0.08465000000001));
#63493=CARTESIAN_POINT('',(-0.0184689851345062,-0.0184241814719618,0.06365));
#63494=CARTESIAN_POINT('',(-0.0211577899118859,-0.0165945500931255,0.06365000000001));
#63495=CARTESIAN_POINT('',(-0.0250405557460001,-0.0139524727409137,0.0591782912689519));
#63496=CARTESIAN_POINT('Origin',(-0.0311262178068916,-0.0144741814719618,
0.06365));
#63497=CARTESIAN_POINT('',(0.0021237821931084,-0.0184241814719618,0.06365));
#63498=CARTESIAN_POINT('',(0.00212378219311841,0.0148536964671725,0.06365000000001));
#63499=CARTESIAN_POINT('',(-0.0158972056958819,-0.0184241814719718,0.06365000000001));
#63500=CARTESIAN_POINT('Origin',(-0.0311262178068916,-0.0144741814719618,
0.08465));
#63501=CARTESIAN_POINT('',(0.0021237821931084,-0.0184241814719618,0.08465));
#63502=CARTESIAN_POINT('',(0.0021237821931184,-0.0184241814719718,0.08465000000001));
#63503=CARTESIAN_POINT('',(0.00212378219311841,0.0148536964671725,0.08465000000001));
#63504=CARTESIAN_POINT('Origin',(0.00212378219310841,0.0148536964671625,
0.08465));
#63505=CARTESIAN_POINT('',(0.0021237821931184,-0.0184241814719718,0.08465000000001));
#63506=CARTESIAN_POINT('Origin',(0.0311237821931084,0.0148536964671625,
0.06865));
#63507=CARTESIAN_POINT('',(0.0311237821931184,-0.0184241814719718,0.06865000000001));
#63508=CARTESIAN_POINT('Origin',(0.00787378219310841,0.0230268185280382,
0.07415));
#63509=CARTESIAN_POINT('',(0.00787378219311841,0.0230268185280482,0.07590000000001));
#63510=CARTESIAN_POINT('',(0.00787378219311841,0.0230268185280482,0.07240000000001));
#63511=CARTESIAN_POINT('Origin',(0.00787378219310841,0.0230268185280382,
0.0759));
#63512=CARTESIAN_POINT('Origin',(0.00787378219310841,0.0230268185280382,
0.0724));
#63513=CARTESIAN_POINT('Origin',(-0.0311262178068916,-0.0184241814719618,
0.06365));
#63514=CARTESIAN_POINT('',(0.00200247846971871,-0.0198416853008431,0.0650675038288813));
#63515=CARTESIAN_POINT('Origin',(0.0311237821931084,-0.0184241814719618,
0.06865));
#63516=CARTESIAN_POINT('',(0.0311237821931184,-0.0184241814719718,0.06865000000001));
#63517=CARTESIAN_POINT('Origin',(0.0293737821931084,-0.0201741814719619,
0.00803151208831422));
#63518=CARTESIAN_POINT('',(0.00756730575344765,-0.0419806579116424,0.0598074230640057));
#63519=CARTESIAN_POINT('Origin',(0.0021237821931084,-0.0184241814719618,
0.08465));
#63520=CARTESIAN_POINT('',(0.00212378219311842,-0.0184241814719718,0.08465000000001));
#63521=CARTESIAN_POINT('Origin',(-0.0158972056958719,-0.0201741814719619,
0.0829));
#107892=UNCERTAINTY_MEASURE_WITH_UNIT(LENGTH_MEASURE(1.E-5),#107911,
'DISTANCE_ACCURACY_VALUE',
'Maximum model space distance between geometric entities at asserted c
onnectivities');
#107898=UNCERTAINTY_MEASURE_WITH_UNIT(LENGTH_MEASURE(1.E-5),#107911,
'DISTANCE_ACCURACY_VALUE',
'Maximum model space distance between geometric entities at asserted c
onnectivities');
#107904=(
GEOMETRIC_REPRESENTATION_CONTEXT(3)
GLOBAL_UNCERTAINTY_ASSIGNED_CONTEXT((#107892))
GLOBAL_UNIT_ASSIGNED_CONTEXT((#107911,#107912,#107913))
REPRESENTATION_CONTEXT('','3D')
);
#107910=(
GEOMETRIC_REPRESENTATION_CONTEXT(3)
GLOBAL_UNCERTAINTY_ASSIGNED_CONTEXT((#107898))
GLOBAL_UNIT_ASSIGNED_CONTEXT((#107911,#107912,#107913))
REPRESENTATION_CONTEXT('','3D')
);
#107911=(
LENGTH_UNIT()
NAMED_UNIT(*)
SI_UNIT($,.METRE.)
);
#107912=(
NAMED_UNIT(*)
PLANE_ANGLE_UNIT()
SI_UNIT($,.RADIAN.)
);
#107913=(
NAMED_UNIT(*)
SI_UNIT($,.STERADIAN.)
SOLID_ANGLE_UNIT()
);
#107919=SHAPE_DEFINITION_REPRESENTATION(#107930,#107951);
#107930=PRODUCT_DEFINITION_SHAPE('',$,#107963);
#107951=SHAPE_REPRESENTATION('',(#45688),#107904);
#107957=PRODUCT_DEFINITION_CONTEXT('part definition',#107992,'design');
#107963=PRODUCT_DEFINITION('Lever','Lever',#107974,#107957);
#107974=PRODUCT_DEFINITION_FORMATION('',$,#107999);
#107992=APPLICATION_CONTEXT('Managed model based 3d engineering');
#107993=PRODUCT_CONTEXT('part definition',#107992,'mechanical');
#107999=PRODUCT('Lever','Lever',
'LEGAL AND USAGE DISCLAIMER: this Data/Model is provided \X2\201C\X0\A
S IS\X2\201D\X0\ for informational and representational only. It is a 
geometric approximation and is NOT engineered, certified, or guarantee
d for dimensional accuracy, exact tolerances, or production-level prec
ision. Vendor disclaims all implied warranties including fitness for a
 particular purpose. DO NOT USE FOR DIRECT PHYSICAL MANUFACTURING, AUT
OMATED PRODUCTION, OR SAFETY-CRITICAL SYSTEMS without independent engi
neering verification and resolution of any design discrepancies.',(#107993));
#108006=PRESENTATION_STYLE_ASSIGNMENT((#108013));
#108013=SURFACE_STYLE_USAGE(.BOTH.,#108020);
#108020=SURFACE_SIDE_STYLE('',(#108027));
#108027=SURFACE_STYLE_FILL_AREA(#108034);
#108034=FILL_AREA_STYLE('Opaque(25,25,25)',(#108041));
#108041=FILL_AREA_STYLE_COLOUR('Opaque(25,25,25)',#108048);
#108048=COLOUR_RGB('Opaque(25,25,25)',0.0980392156862745,0.0980392156862745,
0.0980392156862745);
ENDSEC;
END-ISO-10303-21;
